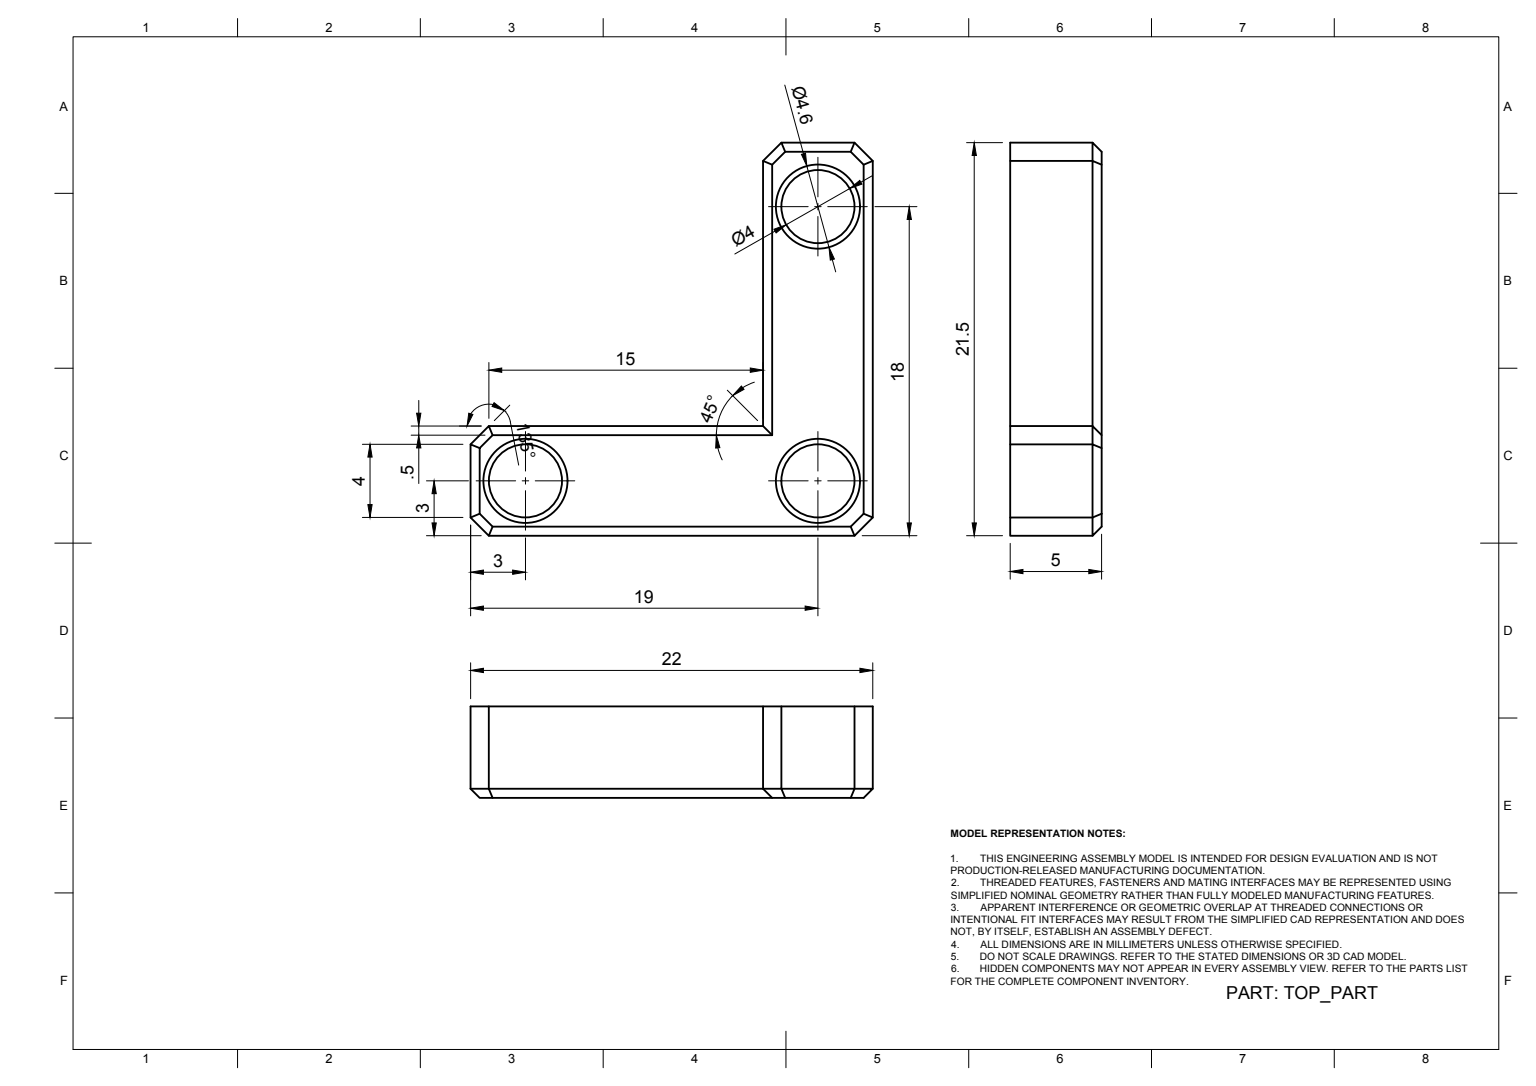
ISO-10303-21;
HEADER;
/* Generated by software containing ST-Developer
 * from STEP Tools, Inc. (www.steptools.com) 
 */

FILE_DESCRIPTION(
/* description */ (''),
/* implementation_level */ '2;1');

FILE_NAME(
/* name */ 'Top_part.step',
/* time_stamp */ '2026-10-04T23:23:09-07:00',
/* author */ (''),
/* organization */ (''),
/* preprocessor_version */ 'ST-DEVELOPER v20.2',
/* originating_system */ 'Autodesk Translation Framework v15.15.0.0',
/* authorisation */ '');

FILE_SCHEMA (('AUTOMOTIVE_DESIGN { 1 0 10303 214 3 1 1 }'));
ENDSEC;

DATA;
#10=MECHANICAL_DESIGN_GEOMETRIC_PRESENTATION_REPRESENTATION('',(#75),#2676);
#56=SHAPE_REPRESENTATION_RELATIONSHIP('SRR','None',#2715,#64);
#64=ADVANCED_BREP_SHAPE_REPRESENTATION('',(#86),#2675);
#75=STYLED_ITEM('',(#2757),#86);
#86=MANIFOLD_SOLID_BREP('Body1',#1486);
#106=CYLINDRICAL_SURFACE('',#1721,2.);
#107=CYLINDRICAL_SURFACE('',#1725,2.);
#108=CYLINDRICAL_SURFACE('',#1753,2.);
#129=FACE_BOUND('',#375,.T.);
#130=FACE_BOUND('',#376,.T.);
#131=FACE_BOUND('',#377,.T.);
#132=FACE_BOUND('',#390,.T.);
#133=FACE_BOUND('',#391,.T.);
#134=FACE_BOUND('',#392,.T.);
#163=PLANE('',#1718);
#164=PLANE('',#1727);
#165=PLANE('',#1728);
#166=PLANE('',#1729);
#167=PLANE('',#1730);
#168=PLANE('',#1731);
#169=PLANE('',#1732);
#170=PLANE('',#1733);
#171=PLANE('',#1734);
#172=PLANE('',#1735);
#173=PLANE('',#1737);
#174=PLANE('',#1738);
#175=PLANE('',#1739);
#176=PLANE('',#1740);
#177=PLANE('',#1741);
#178=PLANE('',#1742);
#179=PLANE('',#1743);
#180=PLANE('',#1744);
#181=PLANE('',#1745);
#182=PLANE('',#1746);
#183=PLANE('',#1747);
#184=PLANE('',#1748);
#185=PLANE('',#1749);
#186=PLANE('',#1750);
#255=FACE_OUTER_BOUND('',#373,.T.);
#256=FACE_OUTER_BOUND('',#374,.T.);
#257=FACE_OUTER_BOUND('',#378,.T.);
#258=FACE_OUTER_BOUND('',#379,.T.);
#259=FACE_OUTER_BOUND('',#380,.T.);
#260=FACE_OUTER_BOUND('',#381,.T.);
#261=FACE_OUTER_BOUND('',#382,.T.);
#262=FACE_OUTER_BOUND('',#383,.T.);
#263=FACE_OUTER_BOUND('',#384,.T.);
#264=FACE_OUTER_BOUND('',#385,.T.);
#265=FACE_OUTER_BOUND('',#386,.T.);
#266=FACE_OUTER_BOUND('',#387,.T.);
#267=FACE_OUTER_BOUND('',#388,.T.);
#268=FACE_OUTER_BOUND('',#389,.T.);
#269=FACE_OUTER_BOUND('',#393,.T.);
#270=FACE_OUTER_BOUND('',#394,.T.);
#271=FACE_OUTER_BOUND('',#395,.T.);
#272=FACE_OUTER_BOUND('',#396,.T.);
#273=FACE_OUTER_BOUND('',#397,.T.);
#274=FACE_OUTER_BOUND('',#398,.T.);
#275=FACE_OUTER_BOUND('',#399,.T.);
#276=FACE_OUTER_BOUND('',#400,.T.);
#277=FACE_OUTER_BOUND('',#401,.T.);
#278=FACE_OUTER_BOUND('',#402,.T.);
#279=FACE_OUTER_BOUND('',#403,.T.);
#280=FACE_OUTER_BOUND('',#404,.T.);
#281=FACE_OUTER_BOUND('',#405,.T.);
#282=FACE_OUTER_BOUND('',#406,.T.);
#283=FACE_OUTER_BOUND('',#407,.T.);
#284=FACE_OUTER_BOUND('',#408,.T.);
#373=EDGE_LOOP('',(#1220,#1221,#1222,#1223));
#374=EDGE_LOOP('',(#1224,#1225,#1226,#1227,#1228,#1229,#1230,#1231,#1232,
#1233,#1234));
#375=EDGE_LOOP('',(#1235));
#376=EDGE_LOOP('',(#1236));
#377=EDGE_LOOP('',(#1237));
#378=EDGE_LOOP('',(#1238,#1239,#1240,#1241));
#379=EDGE_LOOP('',(#1242,#1243,#1244,#1245));
#380=EDGE_LOOP('',(#1246,#1247,#1248,#1249));
#381=EDGE_LOOP('',(#1250,#1251,#1252,#1253));
#382=EDGE_LOOP('',(#1254,#1255,#1256,#1257));
#383=EDGE_LOOP('',(#1258,#1259,#1260,#1261));
#384=EDGE_LOOP('',(#1262,#1263,#1264,#1265));
#385=EDGE_LOOP('',(#1266,#1267,#1268,#1269));
#386=EDGE_LOOP('',(#1270,#1271,#1272,#1273));
#387=EDGE_LOOP('',(#1274,#1275,#1276,#1277));
#388=EDGE_LOOP('',(#1278,#1279,#1280,#1281));
#389=EDGE_LOOP('',(#1282,#1283,#1284,#1285,#1286,#1287,#1288,#1289,#1290,
#1291,#1292));
#390=EDGE_LOOP('',(#1293));
#391=EDGE_LOOP('',(#1294));
#392=EDGE_LOOP('',(#1295));
#393=EDGE_LOOP('',(#1296,#1297,#1298,#1299));
#394=EDGE_LOOP('',(#1300,#1301,#1302,#1303));
#395=EDGE_LOOP('',(#1304,#1305,#1306,#1307));
#396=EDGE_LOOP('',(#1308,#1309,#1310,#1311));
#397=EDGE_LOOP('',(#1312,#1313,#1314,#1315));
#398=EDGE_LOOP('',(#1316,#1317,#1318,#1319));
#399=EDGE_LOOP('',(#1320,#1321,#1322,#1323));
#400=EDGE_LOOP('',(#1324,#1325,#1326,#1327));
#401=EDGE_LOOP('',(#1328,#1329,#1330,#1331));
#402=EDGE_LOOP('',(#1332,#1333,#1334,#1335));
#403=EDGE_LOOP('',(#1336,#1337,#1338,#1339));
#404=EDGE_LOOP('',(#1340,#1341,#1342,#1343));
#405=EDGE_LOOP('',(#1344,#1345,#1346,#1347));
#406=EDGE_LOOP('',(#1348,#1349,#1350,#1351));
#407=EDGE_LOOP('',(#1352,#1353,#1354,#1355));
#408=EDGE_LOOP('',(#1356,#1357,#1358,#1359));
#458=LINE('',#2511,#568);
#459=LINE('',#2516,#569);
#460=LINE('',#2518,#570);
#461=LINE('',#2520,#571);
#462=LINE('',#2522,#572);
#463=LINE('',#2524,#573);
#464=LINE('',#2526,#574);
#465=LINE('',#2528,#575);
#466=LINE('',#2530,#576);
#467=LINE('',#2532,#577);
#468=LINE('',#2534,#578);
#469=LINE('',#2535,#579);
#470=LINE('',#2542,#580);
#471=LINE('',#2547,#581);
#472=LINE('',#2550,#582);
#473=LINE('',#2555,#583);
#474=LINE('',#2556,#584);
#475=LINE('',#2557,#585);
#476=LINE('',#2560,#586);
#477=LINE('',#2561,#587);
#478=LINE('',#2564,#588);
#479=LINE('',#2565,#589);
#480=LINE('',#2568,#590);
#481=LINE('',#2569,#591);
#482=LINE('',#2572,#592);
#483=LINE('',#2574,#593);
#484=LINE('',#2575,#594);
#485=LINE('',#2578,#595);
#486=LINE('',#2579,#596);
#487=LINE('',#2582,#597);
#488=LINE('',#2583,#598);
#489=LINE('',#2586,#599);
#490=LINE('',#2587,#600);
#491=LINE('',#2590,#601);
#492=LINE('',#2592,#602);
#493=LINE('',#2594,#603);
#494=LINE('',#2596,#604);
#495=LINE('',#2598,#605);
#496=LINE('',#2600,#606);
#497=LINE('',#2601,#607);
#498=LINE('',#2606,#608);
#499=LINE('',#2607,#609);
#500=LINE('',#2610,#610);
#501=LINE('',#2612,#611);
#502=LINE('',#2613,#612);
#503=LINE('',#2616,#613);
#504=LINE('',#2617,#614);
#505=LINE('',#2620,#615);
#506=LINE('',#2621,#616);
#507=LINE('',#2624,#617);
#508=LINE('',#2625,#618);
#509=LINE('',#2627,#619);
#510=LINE('',#2629,#620);
#511=LINE('',#2631,#621);
#512=LINE('',#2633,#622);
#513=LINE('',#2635,#623);
#514=LINE('',#2637,#624);
#515=LINE('',#2639,#625);
#516=LINE('',#2641,#626);
#517=LINE('',#2646,#627);
#518=LINE('',#2648,#628);
#568=VECTOR('',#2093,2.15);
#569=VECTOR('',#2098,10.);
#570=VECTOR('',#2099,10.);
#571=VECTOR('',#2100,10.);
#572=VECTOR('',#2101,10.);
#573=VECTOR('',#2102,10.);
#574=VECTOR('',#2103,10.);
#575=VECTOR('',#2104,10.);
#576=VECTOR('',#2105,10.);
#577=VECTOR('',#2106,10.);
#578=VECTOR('',#2107,9.99999999999999);
#579=VECTOR('',#2108,10.);
#580=VECTOR('',#2115,2.);
#581=VECTOR('',#2122,2.15);
#582=VECTOR('',#2125,2.);
#583=VECTOR('',#2130,10.);
#584=VECTOR('',#2131,10.);
#585=VECTOR('',#2132,10.);
#586=VECTOR('',#2135,10.);
#587=VECTOR('',#2136,10.);
#588=VECTOR('',#2139,10.);
#589=VECTOR('',#2140,9.99999999999999);
#590=VECTOR('',#2143,10.);
#591=VECTOR('',#2144,10.);
#592=VECTOR('',#2147,10.);
#593=VECTOR('',#2148,10.);
#594=VECTOR('',#2149,10.);
#595=VECTOR('',#2152,10.);
#596=VECTOR('',#2153,10.);
#597=VECTOR('',#2156,10.);
#598=VECTOR('',#2157,9.99999999999999);
#599=VECTOR('',#2160,10.);
#600=VECTOR('',#2161,10.);
#601=VECTOR('',#2164,10.);
#602=VECTOR('',#2165,10.);
#603=VECTOR('',#2166,10.);
#604=VECTOR('',#2167,10.);
#605=VECTOR('',#2168,10.);
#606=VECTOR('',#2169,10.);
#607=VECTOR('',#2170,10.);
#608=VECTOR('',#2175,10.);
#609=VECTOR('',#2176,10.);
#610=VECTOR('',#2179,10.);
#611=VECTOR('',#2180,10.);
#612=VECTOR('',#2181,10.);
#613=VECTOR('',#2184,10.);
#614=VECTOR('',#2185,10.);
#615=VECTOR('',#2188,10.);
#616=VECTOR('',#2189,10.);
#617=VECTOR('',#2192,10.);
#618=VECTOR('',#2193,10.);
#619=VECTOR('',#2196,10.);
#620=VECTOR('',#2199,10.);
#621=VECTOR('',#2202,10.);
#622=VECTOR('',#2205,10.);
#623=VECTOR('',#2208,10.);
#624=VECTOR('',#2211,10.);
#625=VECTOR('',#2214,10.);
#626=VECTOR('',#2217,10.);
#627=VECTOR('',#2224,2.15);
#628=VECTOR('',#2227,2.);
#691=CIRCLE('',#1716,2.);
#692=CIRCLE('',#1717,2.3);
#693=CIRCLE('',#1719,2.3);
#694=CIRCLE('',#1720,2.3);
#695=CIRCLE('',#1722,2.);
#696=CIRCLE('',#1724,2.);
#697=CIRCLE('',#1726,2.);
#698=CIRCLE('',#1736,2.);
#699=CIRCLE('',#1752,2.);
#775=VERTEX_POINT('',#2508);
#776=VERTEX_POINT('',#2510);
#777=VERTEX_POINT('',#2514);
#778=VERTEX_POINT('',#2515);
#779=VERTEX_POINT('',#2517);
#780=VERTEX_POINT('',#2519);
#781=VERTEX_POINT('',#2521);
#782=VERTEX_POINT('',#2523);
#783=VERTEX_POINT('',#2525);
#784=VERTEX_POINT('',#2527);
#785=VERTEX_POINT('',#2529);
#786=VERTEX_POINT('',#2531);
#787=VERTEX_POINT('',#2533);
#788=VERTEX_POINT('',#2536);
#789=VERTEX_POINT('',#2538);
#790=VERTEX_POINT('',#2541);
#791=VERTEX_POINT('',#2545);
#792=VERTEX_POINT('',#2549);
#793=VERTEX_POINT('',#2553);
#794=VERTEX_POINT('',#2554);
#795=VERTEX_POINT('',#2559);
#796=VERTEX_POINT('',#2563);
#797=VERTEX_POINT('',#2567);
#798=VERTEX_POINT('',#2571);
#799=VERTEX_POINT('',#2573);
#800=VERTEX_POINT('',#2577);
#801=VERTEX_POINT('',#2581);
#802=VERTEX_POINT('',#2585);
#803=VERTEX_POINT('',#2589);
#804=VERTEX_POINT('',#2591);
#805=VERTEX_POINT('',#2593);
#806=VERTEX_POINT('',#2595);
#807=VERTEX_POINT('',#2597);
#808=VERTEX_POINT('',#2599);
#809=VERTEX_POINT('',#2602);
#810=VERTEX_POINT('',#2605);
#811=VERTEX_POINT('',#2609);
#812=VERTEX_POINT('',#2611);
#813=VERTEX_POINT('',#2615);
#814=VERTEX_POINT('',#2619);
#815=VERTEX_POINT('',#2623);
#816=VERTEX_POINT('',#2644);
#928=EDGE_CURVE('',#775,#775,#691,.T.);
#929=EDGE_CURVE('',#775,#776,#458,.T.);
#930=EDGE_CURVE('',#776,#776,#692,.T.);
#931=EDGE_CURVE('',#777,#778,#459,.T.);
#932=EDGE_CURVE('',#779,#777,#460,.T.);
#933=EDGE_CURVE('',#780,#779,#461,.T.);
#934=EDGE_CURVE('',#781,#780,#462,.T.);
#935=EDGE_CURVE('',#782,#781,#463,.T.);
#936=EDGE_CURVE('',#783,#782,#464,.T.);
#937=EDGE_CURVE('',#784,#783,#465,.T.);
#938=EDGE_CURVE('',#785,#784,#466,.T.);
#939=EDGE_CURVE('',#786,#785,#467,.T.);
#940=EDGE_CURVE('',#787,#786,#468,.T.);
#941=EDGE_CURVE('',#778,#787,#469,.T.);
#942=EDGE_CURVE('',#788,#788,#693,.T.);
#943=EDGE_CURVE('',#789,#789,#694,.T.);
#944=EDGE_CURVE('',#775,#790,#470,.T.);
#945=EDGE_CURVE('',#790,#790,#695,.T.);
#946=EDGE_CURVE('',#791,#791,#696,.T.);
#947=EDGE_CURVE('',#791,#788,#471,.T.);
#948=EDGE_CURVE('',#791,#792,#472,.T.);
#949=EDGE_CURVE('',#792,#792,#697,.T.);
#950=EDGE_CURVE('',#793,#794,#473,.T.);
#951=EDGE_CURVE('',#794,#777,#474,.T.);
#952=EDGE_CURVE('',#778,#793,#475,.T.);
#953=EDGE_CURVE('',#787,#795,#476,.T.);
#954=EDGE_CURVE('',#795,#793,#477,.T.);
#955=EDGE_CURVE('',#786,#796,#478,.T.);
#956=EDGE_CURVE('',#796,#795,#479,.T.);
#957=EDGE_CURVE('',#785,#797,#480,.F.);
#958=EDGE_CURVE('',#797,#796,#481,.T.);
#959=EDGE_CURVE('',#793,#798,#482,.T.);
#960=EDGE_CURVE('',#798,#799,#483,.T.);
#961=EDGE_CURVE('',#799,#794,#484,.T.);
#962=EDGE_CURVE('',#800,#795,#485,.T.);
#963=EDGE_CURVE('',#800,#798,#486,.T.);
#964=EDGE_CURVE('',#796,#801,#487,.T.);
#965=EDGE_CURVE('',#801,#800,#488,.T.);
#966=EDGE_CURVE('',#802,#797,#489,.T.);
#967=EDGE_CURVE('',#802,#801,#490,.F.);
#968=EDGE_CURVE('',#803,#802,#491,.T.);
#969=EDGE_CURVE('',#804,#803,#492,.T.);
#970=EDGE_CURVE('',#804,#805,#493,.T.);
#971=EDGE_CURVE('',#806,#805,#494,.T.);
#972=EDGE_CURVE('',#807,#806,#495,.T.);
#973=EDGE_CURVE('',#808,#807,#496,.T.);
#974=EDGE_CURVE('',#799,#808,#497,.F.);
#975=EDGE_CURVE('',#809,#809,#698,.T.);
#976=EDGE_CURVE('',#810,#797,#498,.T.);
#977=EDGE_CURVE('',#784,#810,#499,.T.);
#978=EDGE_CURVE('',#782,#811,#500,.T.);
#979=EDGE_CURVE('',#811,#812,#501,.T.);
#980=EDGE_CURVE('',#812,#783,#502,.T.);
#981=EDGE_CURVE('',#781,#813,#503,.T.);
#982=EDGE_CURVE('',#813,#811,#504,.T.);
#983=EDGE_CURVE('',#780,#814,#505,.T.);
#984=EDGE_CURVE('',#814,#813,#506,.T.);
#985=EDGE_CURVE('',#779,#815,#507,.T.);
#986=EDGE_CURVE('',#815,#814,#508,.T.);
#987=EDGE_CURVE('',#794,#815,#509,.T.);
#988=EDGE_CURVE('',#812,#810,#510,.T.);
#989=EDGE_CURVE('',#803,#810,#511,.T.);
#990=EDGE_CURVE('',#812,#804,#512,.T.);
#991=EDGE_CURVE('',#805,#811,#513,.T.);
#992=EDGE_CURVE('',#813,#806,#514,.T.);
#993=EDGE_CURVE('',#807,#814,#515,.T.);
#994=EDGE_CURVE('',#815,#808,#516,.T.);
#995=EDGE_CURVE('',#816,#816,#699,.T.);
#996=EDGE_CURVE('',#816,#789,#517,.T.);
#997=EDGE_CURVE('',#816,#809,#518,.T.);
#1220=ORIENTED_EDGE('',*,*,#928,.T.);
#1221=ORIENTED_EDGE('',*,*,#929,.T.);
#1222=ORIENTED_EDGE('',*,*,#930,.T.);
#1223=ORIENTED_EDGE('',*,*,#929,.F.);
#1224=ORIENTED_EDGE('',*,*,#931,.F.);
#1225=ORIENTED_EDGE('',*,*,#932,.F.);
#1226=ORIENTED_EDGE('',*,*,#933,.F.);
#1227=ORIENTED_EDGE('',*,*,#934,.F.);
#1228=ORIENTED_EDGE('',*,*,#935,.F.);
#1229=ORIENTED_EDGE('',*,*,#936,.F.);
#1230=ORIENTED_EDGE('',*,*,#937,.F.);
#1231=ORIENTED_EDGE('',*,*,#938,.F.);
#1232=ORIENTED_EDGE('',*,*,#939,.F.);
#1233=ORIENTED_EDGE('',*,*,#940,.F.);
#1234=ORIENTED_EDGE('',*,*,#941,.F.);
#1235=ORIENTED_EDGE('',*,*,#942,.F.);
#1236=ORIENTED_EDGE('',*,*,#943,.F.);
#1237=ORIENTED_EDGE('',*,*,#930,.F.);
#1238=ORIENTED_EDGE('',*,*,#928,.F.);
#1239=ORIENTED_EDGE('',*,*,#944,.T.);
#1240=ORIENTED_EDGE('',*,*,#945,.F.);
#1241=ORIENTED_EDGE('',*,*,#944,.F.);
#1242=ORIENTED_EDGE('',*,*,#946,.T.);
#1243=ORIENTED_EDGE('',*,*,#947,.T.);
#1244=ORIENTED_EDGE('',*,*,#942,.T.);
#1245=ORIENTED_EDGE('',*,*,#947,.F.);
#1246=ORIENTED_EDGE('',*,*,#946,.F.);
#1247=ORIENTED_EDGE('',*,*,#948,.T.);
#1248=ORIENTED_EDGE('',*,*,#949,.F.);
#1249=ORIENTED_EDGE('',*,*,#948,.F.);
#1250=ORIENTED_EDGE('',*,*,#950,.T.);
#1251=ORIENTED_EDGE('',*,*,#951,.T.);
#1252=ORIENTED_EDGE('',*,*,#931,.T.);
#1253=ORIENTED_EDGE('',*,*,#952,.T.);
#1254=ORIENTED_EDGE('',*,*,#941,.T.);
#1255=ORIENTED_EDGE('',*,*,#953,.T.);
#1256=ORIENTED_EDGE('',*,*,#954,.T.);
#1257=ORIENTED_EDGE('',*,*,#952,.F.);
#1258=ORIENTED_EDGE('',*,*,#940,.T.);
#1259=ORIENTED_EDGE('',*,*,#955,.T.);
#1260=ORIENTED_EDGE('',*,*,#956,.T.);
#1261=ORIENTED_EDGE('',*,*,#953,.F.);
#1262=ORIENTED_EDGE('',*,*,#939,.T.);
#1263=ORIENTED_EDGE('',*,*,#957,.T.);
#1264=ORIENTED_EDGE('',*,*,#958,.T.);
#1265=ORIENTED_EDGE('',*,*,#955,.F.);
#1266=ORIENTED_EDGE('',*,*,#950,.F.);
#1267=ORIENTED_EDGE('',*,*,#959,.T.);
#1268=ORIENTED_EDGE('',*,*,#960,.T.);
#1269=ORIENTED_EDGE('',*,*,#961,.T.);
#1270=ORIENTED_EDGE('',*,*,#954,.F.);
#1271=ORIENTED_EDGE('',*,*,#962,.F.);
#1272=ORIENTED_EDGE('',*,*,#963,.T.);
#1273=ORIENTED_EDGE('',*,*,#959,.F.);
#1274=ORIENTED_EDGE('',*,*,#956,.F.);
#1275=ORIENTED_EDGE('',*,*,#964,.T.);
#1276=ORIENTED_EDGE('',*,*,#965,.T.);
#1277=ORIENTED_EDGE('',*,*,#962,.T.);
#1278=ORIENTED_EDGE('',*,*,#958,.F.);
#1279=ORIENTED_EDGE('',*,*,#966,.F.);
#1280=ORIENTED_EDGE('',*,*,#967,.T.);
#1281=ORIENTED_EDGE('',*,*,#964,.F.);
#1282=ORIENTED_EDGE('',*,*,#965,.F.);
#1283=ORIENTED_EDGE('',*,*,#967,.F.);
#1284=ORIENTED_EDGE('',*,*,#968,.F.);
#1285=ORIENTED_EDGE('',*,*,#969,.F.);
#1286=ORIENTED_EDGE('',*,*,#970,.T.);
#1287=ORIENTED_EDGE('',*,*,#971,.F.);
#1288=ORIENTED_EDGE('',*,*,#972,.F.);
#1289=ORIENTED_EDGE('',*,*,#973,.F.);
#1290=ORIENTED_EDGE('',*,*,#974,.F.);
#1291=ORIENTED_EDGE('',*,*,#960,.F.);
#1292=ORIENTED_EDGE('',*,*,#963,.F.);
#1293=ORIENTED_EDGE('',*,*,#945,.T.);
#1294=ORIENTED_EDGE('',*,*,#949,.T.);
#1295=ORIENTED_EDGE('',*,*,#975,.T.);
#1296=ORIENTED_EDGE('',*,*,#976,.T.);
#1297=ORIENTED_EDGE('',*,*,#957,.F.);
#1298=ORIENTED_EDGE('',*,*,#938,.T.);
#1299=ORIENTED_EDGE('',*,*,#977,.T.);
#1300=ORIENTED_EDGE('',*,*,#936,.T.);
#1301=ORIENTED_EDGE('',*,*,#978,.T.);
#1302=ORIENTED_EDGE('',*,*,#979,.T.);
#1303=ORIENTED_EDGE('',*,*,#980,.T.);
#1304=ORIENTED_EDGE('',*,*,#935,.T.);
#1305=ORIENTED_EDGE('',*,*,#981,.T.);
#1306=ORIENTED_EDGE('',*,*,#982,.T.);
#1307=ORIENTED_EDGE('',*,*,#978,.F.);
#1308=ORIENTED_EDGE('',*,*,#934,.T.);
#1309=ORIENTED_EDGE('',*,*,#983,.T.);
#1310=ORIENTED_EDGE('',*,*,#984,.T.);
#1311=ORIENTED_EDGE('',*,*,#981,.F.);
#1312=ORIENTED_EDGE('',*,*,#933,.T.);
#1313=ORIENTED_EDGE('',*,*,#985,.T.);
#1314=ORIENTED_EDGE('',*,*,#986,.T.);
#1315=ORIENTED_EDGE('',*,*,#983,.F.);
#1316=ORIENTED_EDGE('',*,*,#951,.F.);
#1317=ORIENTED_EDGE('',*,*,#987,.T.);
#1318=ORIENTED_EDGE('',*,*,#985,.F.);
#1319=ORIENTED_EDGE('',*,*,#932,.T.);
#1320=ORIENTED_EDGE('',*,*,#937,.T.);
#1321=ORIENTED_EDGE('',*,*,#980,.F.);
#1322=ORIENTED_EDGE('',*,*,#988,.T.);
#1323=ORIENTED_EDGE('',*,*,#977,.F.);
#1324=ORIENTED_EDGE('',*,*,#976,.F.);
#1325=ORIENTED_EDGE('',*,*,#989,.F.);
#1326=ORIENTED_EDGE('',*,*,#968,.T.);
#1327=ORIENTED_EDGE('',*,*,#966,.T.);
#1328=ORIENTED_EDGE('',*,*,#988,.F.);
#1329=ORIENTED_EDGE('',*,*,#990,.T.);
#1330=ORIENTED_EDGE('',*,*,#969,.T.);
#1331=ORIENTED_EDGE('',*,*,#989,.T.);
#1332=ORIENTED_EDGE('',*,*,#979,.F.);
#1333=ORIENTED_EDGE('',*,*,#991,.F.);
#1334=ORIENTED_EDGE('',*,*,#970,.F.);
#1335=ORIENTED_EDGE('',*,*,#990,.F.);
#1336=ORIENTED_EDGE('',*,*,#982,.F.);
#1337=ORIENTED_EDGE('',*,*,#992,.T.);
#1338=ORIENTED_EDGE('',*,*,#971,.T.);
#1339=ORIENTED_EDGE('',*,*,#991,.T.);
#1340=ORIENTED_EDGE('',*,*,#984,.F.);
#1341=ORIENTED_EDGE('',*,*,#993,.F.);
#1342=ORIENTED_EDGE('',*,*,#972,.T.);
#1343=ORIENTED_EDGE('',*,*,#992,.F.);
#1344=ORIENTED_EDGE('',*,*,#986,.F.);
#1345=ORIENTED_EDGE('',*,*,#994,.T.);
#1346=ORIENTED_EDGE('',*,*,#973,.T.);
#1347=ORIENTED_EDGE('',*,*,#993,.T.);
#1348=ORIENTED_EDGE('',*,*,#987,.F.);
#1349=ORIENTED_EDGE('',*,*,#961,.F.);
#1350=ORIENTED_EDGE('',*,*,#974,.T.);
#1351=ORIENTED_EDGE('',*,*,#994,.F.);
#1352=ORIENTED_EDGE('',*,*,#995,.T.);
#1353=ORIENTED_EDGE('',*,*,#996,.T.);
#1354=ORIENTED_EDGE('',*,*,#943,.T.);
#1355=ORIENTED_EDGE('',*,*,#996,.F.);
#1356=ORIENTED_EDGE('',*,*,#995,.F.);
#1357=ORIENTED_EDGE('',*,*,#997,.T.);
#1358=ORIENTED_EDGE('',*,*,#975,.F.);
#1359=ORIENTED_EDGE('',*,*,#997,.F.);
#1375=CONICAL_SURFACE('',#1715,2.15,0.785398163397448);
#1376=CONICAL_SURFACE('',#1723,2.15,0.785398163397448);
#1377=CONICAL_SURFACE('',#1751,2.15,0.785398163397448);
#1446=ADVANCED_FACE('',(#255),#1375,.F.);
#1447=ADVANCED_FACE('',(#256,#129,#130,#131),#163,.T.);
#1448=ADVANCED_FACE('',(#257),#106,.F.);
#1449=ADVANCED_FACE('',(#258),#1376,.F.);
#1450=ADVANCED_FACE('',(#259),#107,.F.);
#1451=ADVANCED_FACE('',(#260),#164,.T.);
#1452=ADVANCED_FACE('',(#261),#165,.T.);
#1453=ADVANCED_FACE('',(#262),#166,.T.);
#1454=ADVANCED_FACE('',(#263),#167,.T.);
#1455=ADVANCED_FACE('',(#264),#168,.T.);
#1456=ADVANCED_FACE('',(#265),#169,.T.);
#1457=ADVANCED_FACE('',(#266),#170,.T.);
#1458=ADVANCED_FACE('',(#267),#171,.T.);
#1459=ADVANCED_FACE('',(#268,#132,#133,#134),#172,.F.);
#1460=ADVANCED_FACE('',(#269),#173,.T.);
#1461=ADVANCED_FACE('',(#270),#174,.T.);
#1462=ADVANCED_FACE('',(#271),#175,.T.);
#1463=ADVANCED_FACE('',(#272),#176,.T.);
#1464=ADVANCED_FACE('',(#273),#177,.T.);
#1465=ADVANCED_FACE('',(#274),#178,.T.);
#1466=ADVANCED_FACE('',(#275),#179,.T.);
#1467=ADVANCED_FACE('',(#276),#180,.T.);
#1468=ADVANCED_FACE('',(#277),#181,.T.);
#1469=ADVANCED_FACE('',(#278),#182,.T.);
#1470=ADVANCED_FACE('',(#279),#183,.T.);
#1471=ADVANCED_FACE('',(#280),#184,.T.);
#1472=ADVANCED_FACE('',(#281),#185,.T.);
#1473=ADVANCED_FACE('',(#282),#186,.T.);
#1474=ADVANCED_FACE('',(#283),#1377,.F.);
#1475=ADVANCED_FACE('',(#284),#108,.F.);
#1486=CLOSED_SHELL('',(#1446,#1447,#1448,#1449,#1450,#1451,#1452,#1453,
#1454,#1455,#1456,#1457,#1458,#1459,#1460,#1461,#1462,#1463,#1464,#1465,
#1466,#1467,#1468,#1469,#1470,#1471,#1472,#1473,#1474,#1475));
#1714=AXIS2_PLACEMENT_3D('',#2506,#2087,#2088);
#1715=AXIS2_PLACEMENT_3D('',#2507,#2089,#2090);
#1716=AXIS2_PLACEMENT_3D('',#2509,#2091,#2092);
#1717=AXIS2_PLACEMENT_3D('',#2512,#2094,#2095);
#1718=AXIS2_PLACEMENT_3D('',#2513,#2096,#2097);
#1719=AXIS2_PLACEMENT_3D('',#2537,#2109,#2110);
#1720=AXIS2_PLACEMENT_3D('',#2539,#2111,#2112);
#1721=AXIS2_PLACEMENT_3D('',#2540,#2113,#2114);
#1722=AXIS2_PLACEMENT_3D('',#2543,#2116,#2117);
#1723=AXIS2_PLACEMENT_3D('',#2544,#2118,#2119);
#1724=AXIS2_PLACEMENT_3D('',#2546,#2120,#2121);
#1725=AXIS2_PLACEMENT_3D('',#2548,#2123,#2124);
#1726=AXIS2_PLACEMENT_3D('',#2551,#2126,#2127);
#1727=AXIS2_PLACEMENT_3D('',#2552,#2128,#2129);
#1728=AXIS2_PLACEMENT_3D('',#2558,#2133,#2134);
#1729=AXIS2_PLACEMENT_3D('',#2562,#2137,#2138);
#1730=AXIS2_PLACEMENT_3D('',#2566,#2141,#2142);
#1731=AXIS2_PLACEMENT_3D('',#2570,#2145,#2146);
#1732=AXIS2_PLACEMENT_3D('',#2576,#2150,#2151);
#1733=AXIS2_PLACEMENT_3D('',#2580,#2154,#2155);
#1734=AXIS2_PLACEMENT_3D('',#2584,#2158,#2159);
#1735=AXIS2_PLACEMENT_3D('',#2588,#2162,#2163);
#1736=AXIS2_PLACEMENT_3D('',#2603,#2171,#2172);
#1737=AXIS2_PLACEMENT_3D('',#2604,#2173,#2174);
#1738=AXIS2_PLACEMENT_3D('',#2608,#2177,#2178);
#1739=AXIS2_PLACEMENT_3D('',#2614,#2182,#2183);
#1740=AXIS2_PLACEMENT_3D('',#2618,#2186,#2187);
#1741=AXIS2_PLACEMENT_3D('',#2622,#2190,#2191);
#1742=AXIS2_PLACEMENT_3D('',#2626,#2194,#2195);
#1743=AXIS2_PLACEMENT_3D('',#2628,#2197,#2198);
#1744=AXIS2_PLACEMENT_3D('',#2630,#2200,#2201);
#1745=AXIS2_PLACEMENT_3D('',#2632,#2203,#2204);
#1746=AXIS2_PLACEMENT_3D('',#2634,#2206,#2207);
#1747=AXIS2_PLACEMENT_3D('',#2636,#2209,#2210);
#1748=AXIS2_PLACEMENT_3D('',#2638,#2212,#2213);
#1749=AXIS2_PLACEMENT_3D('',#2640,#2215,#2216);
#1750=AXIS2_PLACEMENT_3D('',#2642,#2218,#2219);
#1751=AXIS2_PLACEMENT_3D('',#2643,#2220,#2221);
#1752=AXIS2_PLACEMENT_3D('',#2645,#2222,#2223);
#1753=AXIS2_PLACEMENT_3D('',#2647,#2225,#2226);
#2087=DIRECTION('axis',(0.,0.,1.));
#2088=DIRECTION('refdir',(1.,0.,0.));
#2089=DIRECTION('center_axis',(0.,0.,1.));
#2090=DIRECTION('ref_axis',(-1.,0.,0.));
#2091=DIRECTION('center_axis',(0.,0.,-1.));
#2092=DIRECTION('ref_axis',(-1.,0.,0.));
#2093=DIRECTION('',(0.707106781186547,8.65956056235493E-17,0.707106781186548));
#2094=DIRECTION('center_axis',(0.,0.,1.));
#2095=DIRECTION('ref_axis',(-1.,0.,0.));
#2096=DIRECTION('center_axis',(0.,0.,1.));
#2097=DIRECTION('ref_axis',(1.,0.,0.));
#2098=DIRECTION('',(-0.707106781186548,0.707106781186547,0.));
#2099=DIRECTION('',(-1.,0.,0.));
#2100=DIRECTION('',(-0.707106781186548,-0.707106781186547,0.));
#2101=DIRECTION('',(0.,-1.,0.));
#2102=DIRECTION('',(0.707106781186547,-0.707106781186547,0.));
#2103=DIRECTION('',(1.,0.,0.));
#2104=DIRECTION('',(0.707106781186547,0.707106781186548,0.));
#2105=DIRECTION('',(0.,1.,0.));
#2106=DIRECTION('',(1.,0.,0.));
#2107=DIRECTION('',(0.707106781186548,0.707106781186547,0.));
#2108=DIRECTION('',(0.,1.,0.));
#2109=DIRECTION('center_axis',(0.,0.,1.));
#2110=DIRECTION('ref_axis',(-1.,0.,0.));
#2111=DIRECTION('center_axis',(0.,0.,1.));
#2112=DIRECTION('ref_axis',(-1.,0.,0.));
#2113=DIRECTION('center_axis',(0.,0.,-1.));
#2114=DIRECTION('ref_axis',(-1.,0.,0.));
#2115=DIRECTION('',(0.,0.,-1.));
#2116=DIRECTION('center_axis',(0.,0.,1.));
#2117=DIRECTION('ref_axis',(-1.,0.,0.));
#2118=DIRECTION('center_axis',(0.,0.,1.));
#2119=DIRECTION('ref_axis',(-1.,0.,0.));
#2120=DIRECTION('center_axis',(0.,0.,-1.));
#2121=DIRECTION('ref_axis',(-1.,0.,0.));
#2122=DIRECTION('',(0.707106781186547,8.65956056235493E-17,0.707106781186548));
#2123=DIRECTION('center_axis',(0.,0.,-1.));
#2124=DIRECTION('ref_axis',(-1.,0.,0.));
#2125=DIRECTION('',(0.,0.,-1.));
#2126=DIRECTION('center_axis',(0.,0.,1.));
#2127=DIRECTION('ref_axis',(-1.,0.,0.));
#2128=DIRECTION('center_axis',(-0.500000000000001,-0.500000000000001,0.707106781186546));
#2129=DIRECTION('ref_axis',(0.816496580927725,-1.47935320064922E-16,0.577350269189627));
#2130=DIRECTION('',(0.707106781186548,-0.707106781186547,0.));
#2131=DIRECTION('',(0.281084637714816,0.678598344545848,0.678598344545848));
#2132=DIRECTION('',(-0.678598344545848,-0.281084637714818,-0.678598344545848));
#2133=DIRECTION('center_axis',(-0.707106781186548,0.,0.707106781186548));
#2134=DIRECTION('ref_axis',(0.707106781186548,0.,0.707106781186548));
#2135=DIRECTION('',(-0.678598344545847,0.281084637714821,-0.678598344545847));
#2136=DIRECTION('',(0.,-1.,0.));
#2137=DIRECTION('center_axis',(-0.5,0.500000000000001,0.707106781186547));
#2138=DIRECTION('ref_axis',(0.816496580927726,1.11022302462516E-16,0.577350269189626));
#2139=DIRECTION('',(-0.281084637714819,0.678598344545847,-0.678598344545848));
#2140=DIRECTION('',(-0.707106781186548,-0.707106781186547,0.));
#2141=DIRECTION('center_axis',(0.,0.707106781186548,0.707106781186547));
#2142=DIRECTION('ref_axis',(1.,0.,0.));
#2143=DIRECTION('',(0.577350269189626,-0.577350269189625,0.577350269189626));
#2144=DIRECTION('',(-1.,0.,0.));
#2145=DIRECTION('center_axis',(-0.707106781186547,-0.707106781186548,0.));
#2146=DIRECTION('ref_axis',(0.,0.,1.));
#2147=DIRECTION('',(0.,0.,-1.));
#2148=DIRECTION('',(0.707106781186548,-0.707106781186547,0.));
#2149=DIRECTION('',(0.,0.,1.));
#2150=DIRECTION('center_axis',(-1.,0.,0.));
#2151=DIRECTION('ref_axis',(0.,-1.,0.));
#2152=DIRECTION('',(0.,0.,1.));
#2153=DIRECTION('',(0.,-1.,0.));
#2154=DIRECTION('center_axis',(-0.707106781186547,0.707106781186549,0.));
#2155=DIRECTION('ref_axis',(0.,0.,1.));
#2156=DIRECTION('',(0.,0.,-1.));
#2157=DIRECTION('',(-0.707106781186548,-0.707106781186547,0.));
#2158=DIRECTION('center_axis',(0.,1.,0.));
#2159=DIRECTION('ref_axis',(-1.,0.,0.));
#2160=DIRECTION('',(0.,0.,1.));
#2161=DIRECTION('',(1.,0.,0.));
#2162=DIRECTION('center_axis',(0.,0.,1.));
#2163=DIRECTION('ref_axis',(1.,0.,0.));
#2164=DIRECTION('',(0.,-1.,0.));
#2165=DIRECTION('',(-0.707106781186547,-0.707106781186548,0.));
#2166=DIRECTION('',(1.,0.,0.));
#2167=DIRECTION('',(-0.707106781186547,0.707106781186547,0.));
#2168=DIRECTION('',(0.,1.,0.));
#2169=DIRECTION('',(0.707106781186548,0.707106781186547,0.));
#2170=DIRECTION('',(-1.,0.,0.));
#2171=DIRECTION('center_axis',(0.,0.,1.));
#2172=DIRECTION('ref_axis',(-1.,0.,0.));
#2173=DIRECTION('center_axis',(-0.707106781186548,0.,0.707106781186548));
#2174=DIRECTION('ref_axis',(0.707106781186548,0.,0.707106781186548));
#2175=DIRECTION('',(0.,-1.,0.));
#2176=DIRECTION('',(-0.678598344545848,0.281084637714819,-0.678598344545847));
#2177=DIRECTION('center_axis',(0.,0.707106781186548,0.707106781186548));
#2178=DIRECTION('ref_axis',(1.,0.,0.));
#2179=DIRECTION('',(0.281084637714818,0.678598344545848,-0.678598344545848));
#2180=DIRECTION('',(-1.,0.,0.));
#2181=DIRECTION('',(0.281084637714822,-0.678598344545847,0.678598344545847));
#2182=DIRECTION('center_axis',(0.500000000000001,0.500000000000001,0.707106781186547));
#2183=DIRECTION('ref_axis',(0.816496580927725,1.16630067516701E-16,-0.577350269189627));
#2184=DIRECTION('',(0.678598344545847,0.281084637714819,-0.678598344545847));
#2185=DIRECTION('',(-0.707106781186547,0.707106781186547,0.));
#2186=DIRECTION('center_axis',(0.707106781186548,0.,0.707106781186548));
#2187=DIRECTION('ref_axis',(0.707106781186548,0.,-0.707106781186548));
#2188=DIRECTION('',(0.678598344545847,-0.281084637714821,-0.678598344545847));
#2189=DIRECTION('',(0.,1.,0.));
#2190=DIRECTION('center_axis',(0.5,-0.500000000000001,0.707106781186547));
#2191=DIRECTION('ref_axis',(0.816496580927726,1.11022302462516E-16,-0.577350269189626));
#2192=DIRECTION('',(0.281084637714819,-0.678598344545847,-0.678598344545847));
#2193=DIRECTION('',(0.707106781186548,0.707106781186547,0.));
#2194=DIRECTION('center_axis',(0.,-0.707106781186548,0.707106781186548));
#2195=DIRECTION('ref_axis',(1.,0.,0.));
#2196=DIRECTION('',(1.,0.,0.));
#2197=DIRECTION('center_axis',(-0.500000000000001,0.5,0.707106781186547));
#2198=DIRECTION('ref_axis',(0.816496580927725,-1.19433950043794E-16,0.577350269189627));
#2199=DIRECTION('',(-0.707106781186547,-0.707106781186548,0.));
#2200=DIRECTION('center_axis',(-1.,0.,0.));
#2201=DIRECTION('ref_axis',(0.,-1.,0.));
#2202=DIRECTION('',(0.,0.,1.));
#2203=DIRECTION('center_axis',(-0.707106781186548,0.707106781186547,0.));
#2204=DIRECTION('ref_axis',(0.,0.,1.));
#2205=DIRECTION('',(0.,0.,-1.));
#2206=DIRECTION('center_axis',(0.,1.,0.));
#2207=DIRECTION('ref_axis',(-1.,0.,0.));
#2208=DIRECTION('',(0.,0.,1.));
#2209=DIRECTION('center_axis',(0.707106781186548,0.707106781186548,0.));
#2210=DIRECTION('ref_axis',(0.,0.,-1.));
#2211=DIRECTION('',(0.,0.,-1.));
#2212=DIRECTION('center_axis',(1.,0.,0.));
#2213=DIRECTION('ref_axis',(0.,1.,0.));
#2214=DIRECTION('',(0.,0.,1.));
#2215=DIRECTION('center_axis',(0.707106781186547,-0.707106781186548,0.));
#2216=DIRECTION('ref_axis',(0.,0.,-1.));
#2217=DIRECTION('',(0.,0.,-1.));
#2218=DIRECTION('center_axis',(0.,-1.,0.));
#2219=DIRECTION('ref_axis',(1.,0.,0.));
#2220=DIRECTION('center_axis',(0.,0.,1.));
#2221=DIRECTION('ref_axis',(-1.,0.,0.));
#2222=DIRECTION('center_axis',(0.,0.,-1.));
#2223=DIRECTION('ref_axis',(-1.,0.,0.));
#2224=DIRECTION('',(0.707106781186547,8.65956056235493E-17,0.707106781186548));
#2225=DIRECTION('center_axis',(0.,0.,-1.));
#2226=DIRECTION('ref_axis',(-1.,0.,0.));
#2227=DIRECTION('',(0.,0.,-1.));
#2506=CARTESIAN_POINT('',(0.,0.,0.));
#2507=CARTESIAN_POINT('Origin',(-8.,-7.5,12.35));
#2508=CARTESIAN_POINT('',(-6.,-7.5,12.2));
#2509=CARTESIAN_POINT('Origin',(-8.,-7.5,12.2));
#2510=CARTESIAN_POINT('',(-5.7,-7.5,12.5));
#2511=CARTESIAN_POINT('',(-5.85,-7.5,12.35));
#2512=CARTESIAN_POINT('Origin',(-8.,-7.5,12.5));
#2513=CARTESIAN_POINT('Origin',(0.,0.,12.5));
#2514=CARTESIAN_POINT('',(-9.79289321881345,-10.,12.5));
#2515=CARTESIAN_POINT('',(-10.5,-9.29289321881345,12.5));
#2516=CARTESIAN_POINT('',(-10.0214466094067,-9.77144660940673,12.5));
#2517=CARTESIAN_POINT('',(9.79289321881345,-10.,12.5));
#2518=CARTESIAN_POINT('',(-5.5,-10.,12.5));
#2519=CARTESIAN_POINT('',(10.5,-9.29289321881345,12.5));
#2520=CARTESIAN_POINT('',(10.0214466094067,-9.77144660940673,12.5));
#2521=CARTESIAN_POINT('',(10.5,9.79289321881345,12.5));
#2522=CARTESIAN_POINT('',(10.5,-5.5,12.5));
#2523=CARTESIAN_POINT('',(9.79289321881345,10.5,12.5));
#2524=CARTESIAN_POINT('',(10.1464466094067,10.1464466094067,12.5));
#2525=CARTESIAN_POINT('',(6.20710678118655,10.5,12.5));
#2526=CARTESIAN_POINT('',(5.5,10.5,12.5));
#2527=CARTESIAN_POINT('',(5.5,9.79289321881345,12.5));
#2528=CARTESIAN_POINT('',(1.85355339059327,6.14644660940672,12.5));
#2529=CARTESIAN_POINT('',(5.5,-5.,12.5));
#2530=CARTESIAN_POINT('',(5.5,5.5,12.5));
#2531=CARTESIAN_POINT('',(-9.79289321881345,-5.,12.5));
#2532=CARTESIAN_POINT('',(2.5,-5.,12.5));
#2533=CARTESIAN_POINT('',(-10.5,-5.70710678118654,12.5));
#2534=CARTESIAN_POINT('',(-6.27144660940672,-1.47855339059328,12.5));
#2535=CARTESIAN_POINT('',(-10.5,-2.5,12.5));
#2536=CARTESIAN_POINT('',(10.3,-7.5,12.5));
#2537=CARTESIAN_POINT('Origin',(8.,-7.5,12.5));
#2538=CARTESIAN_POINT('',(10.3,7.5,12.5));
#2539=CARTESIAN_POINT('Origin',(8.,7.5,12.5));
#2540=CARTESIAN_POINT('Origin',(-8.,-7.5,12.5));
#2541=CARTESIAN_POINT('',(-6.,-7.5,7.5));
#2542=CARTESIAN_POINT('',(-6.,-7.5,12.5));
#2543=CARTESIAN_POINT('Origin',(-8.,-7.5,7.5));
#2544=CARTESIAN_POINT('Origin',(8.,-7.5,12.35));
#2545=CARTESIAN_POINT('',(10.,-7.5,12.2));
#2546=CARTESIAN_POINT('Origin',(8.,-7.5,12.2));
#2547=CARTESIAN_POINT('',(10.15,-7.5,12.35));
#2548=CARTESIAN_POINT('Origin',(8.,-7.5,12.5));
#2549=CARTESIAN_POINT('',(10.,-7.5,7.5));
#2550=CARTESIAN_POINT('',(10.,-7.5,12.5));
#2551=CARTESIAN_POINT('Origin',(8.,-7.5,7.5));
#2552=CARTESIAN_POINT('Origin',(-10.1982233047034,-9.94822330470336,12.25));
#2553=CARTESIAN_POINT('',(-11.,-9.5,12.));
#2554=CARTESIAN_POINT('',(-10.,-10.5,12.));
#2555=CARTESIAN_POINT('',(-10.375,-10.125,12.));
#2556=CARTESIAN_POINT('',(-9.7059086127755,-9.7900005843855,12.7099994156145));
#2557=CARTESIAN_POINT('',(-10.5,-9.29289321881345,12.5));
#2558=CARTESIAN_POINT('Origin',(-10.75,-2.5,12.25));
#2559=CARTESIAN_POINT('',(-11.,-5.5,12.));
#2560=CARTESIAN_POINT('',(-10.5,-5.70710678118654,12.5));
#2561=CARTESIAN_POINT('',(-11.,-2.5,12.));
#2562=CARTESIAN_POINT('Origin',(-6.44822330470336,-1.30177669529664,12.25));
#2563=CARTESIAN_POINT('',(-10.,-4.5,12.));
#2564=CARTESIAN_POINT('',(-9.79289321881345,-5.,12.5));
#2565=CARTESIAN_POINT('',(-6.62499999999999,-1.125,12.));
#2566=CARTESIAN_POINT('Origin',(2.5,-4.75,12.25));
#2567=CARTESIAN_POINT('',(5.,-4.5,12.));
#2568=CARTESIAN_POINT('',(3.08333333333333,-2.58333333333333,10.0833333333333));
#2569=CARTESIAN_POINT('',(2.5,-4.5,12.));
#2570=CARTESIAN_POINT('Origin',(-10.5,-10.,7.5));
#2571=CARTESIAN_POINT('',(-11.,-9.5,7.5));
#2572=CARTESIAN_POINT('',(-11.,-9.5,7.5));
#2573=CARTESIAN_POINT('',(-10.,-10.5,7.5));
#2574=CARTESIAN_POINT('',(-10.375,-10.125,7.5));
#2575=CARTESIAN_POINT('',(-10.,-10.5,7.5));
#2576=CARTESIAN_POINT('Origin',(-11.,-5.,7.5));
#2577=CARTESIAN_POINT('',(-11.,-5.5,7.5));
#2578=CARTESIAN_POINT('',(-11.,-5.5,7.5));
#2579=CARTESIAN_POINT('',(-11.,8.,7.5));
#2580=CARTESIAN_POINT('Origin',(-10.5,-5.,7.5));
#2581=CARTESIAN_POINT('',(-10.,-4.5,7.5));
#2582=CARTESIAN_POINT('',(-10.,-4.5,7.5));
#2583=CARTESIAN_POINT('',(-6.62499999999999,-1.125,7.5));
#2584=CARTESIAN_POINT('Origin',(5.,-4.5,7.5));
#2585=CARTESIAN_POINT('',(5.,-4.5,7.5));
#2586=CARTESIAN_POINT('',(5.,-4.5,7.5));
#2587=CARTESIAN_POINT('',(2.5,-4.5,7.5));
#2588=CARTESIAN_POINT('Origin',(0.,0.,7.5));
#2589=CARTESIAN_POINT('',(5.,10.,7.5));
#2590=CARTESIAN_POINT('',(5.,11.,7.5));
#2591=CARTESIAN_POINT('',(6.,11.,7.5));
#2592=CARTESIAN_POINT('',(1.5,6.5,7.5));
#2593=CARTESIAN_POINT('',(10.,11.,7.5));
#2594=CARTESIAN_POINT('',(5.,11.,7.5));
#2595=CARTESIAN_POINT('',(11.,10.,7.5));
#2596=CARTESIAN_POINT('',(10.5,10.5,7.5));
#2597=CARTESIAN_POINT('',(11.,-9.5,7.5));
#2598=CARTESIAN_POINT('',(11.,-11.,7.5));
#2599=CARTESIAN_POINT('',(10.,-10.5,7.5));
#2600=CARTESIAN_POINT('',(10.375,-10.125,7.5));
#2601=CARTESIAN_POINT('',(-5.5,-10.5,7.5));
#2602=CARTESIAN_POINT('',(10.,7.5,7.5));
#2603=CARTESIAN_POINT('Origin',(8.,7.5,7.5));
#2604=CARTESIAN_POINT('Origin',(5.25,5.5,12.25));
#2605=CARTESIAN_POINT('',(5.,10.,12.));
#2606=CARTESIAN_POINT('',(5.,5.5,12.));
#2607=CARTESIAN_POINT('',(5.5,9.79289321881345,12.5));
#2608=CARTESIAN_POINT('Origin',(5.5,10.75,12.25));
#2609=CARTESIAN_POINT('',(10.,11.,12.));
#2610=CARTESIAN_POINT('',(9.79289321881345,10.5,12.5));
#2611=CARTESIAN_POINT('',(6.,11.,12.));
#2612=CARTESIAN_POINT('',(5.5,11.,12.));
#2613=CARTESIAN_POINT('',(6.,11.,12.));
#2614=CARTESIAN_POINT('Origin',(10.3232233047034,10.3232233047034,12.25));
#2615=CARTESIAN_POINT('',(11.,10.,12.));
#2616=CARTESIAN_POINT('',(10.5,9.79289321881345,12.5));
#2617=CARTESIAN_POINT('',(10.5,10.5,12.));
#2618=CARTESIAN_POINT('Origin',(10.75,-5.5,12.25));
#2619=CARTESIAN_POINT('',(11.,-9.5,12.));
#2620=CARTESIAN_POINT('',(10.5,-9.29289321881345,12.5));
#2621=CARTESIAN_POINT('',(11.,-5.5,12.));
#2622=CARTESIAN_POINT('Origin',(10.1982233047034,-9.94822330470337,12.25));
#2623=CARTESIAN_POINT('',(10.,-10.5,12.));
#2624=CARTESIAN_POINT('',(9.79289321881345,-10.,12.5));
#2625=CARTESIAN_POINT('',(10.375,-10.125,12.));
#2626=CARTESIAN_POINT('Origin',(-5.5,-10.25,12.25));
#2627=CARTESIAN_POINT('',(-5.5,-10.5,12.));
#2628=CARTESIAN_POINT('Origin',(1.67677669529664,6.32322330470336,12.25));
#2629=CARTESIAN_POINT('',(1.5,6.5,12.));
#2630=CARTESIAN_POINT('Origin',(5.,11.,7.5));
#2631=CARTESIAN_POINT('',(5.,10.,7.5));
#2632=CARTESIAN_POINT('Origin',(5.5,10.5,7.5));
#2633=CARTESIAN_POINT('',(6.,11.,7.5));
#2634=CARTESIAN_POINT('Origin',(11.,11.,7.5));
#2635=CARTESIAN_POINT('',(10.,11.,7.5));
#2636=CARTESIAN_POINT('Origin',(10.5,10.5,7.5));
#2637=CARTESIAN_POINT('',(11.,10.,7.5));
#2638=CARTESIAN_POINT('Origin',(11.,-11.,7.5));
#2639=CARTESIAN_POINT('',(11.,-9.5,7.5));
#2640=CARTESIAN_POINT('Origin',(10.5,-10.,7.5));
#2641=CARTESIAN_POINT('',(10.,-10.5,7.5));
#2642=CARTESIAN_POINT('Origin',(-11.,-10.5,7.5));
#2643=CARTESIAN_POINT('Origin',(8.,7.5,12.35));
#2644=CARTESIAN_POINT('',(10.,7.5,12.2));
#2645=CARTESIAN_POINT('Origin',(8.,7.5,12.2));
#2646=CARTESIAN_POINT('',(10.15,7.5,12.35));
#2647=CARTESIAN_POINT('Origin',(8.,7.5,12.5));
#2648=CARTESIAN_POINT('',(10.,7.5,12.5));
#2665=UNCERTAINTY_MEASURE_WITH_UNIT(LENGTH_MEASURE(0.01),#2677,
'DISTANCE_ACCURACY_VALUE',
'Maximum model space distance between geometric entities at asserted c
onnectivities');
#2666=UNCERTAINTY_MEASURE_WITH_UNIT(LENGTH_MEASURE(0.01),#2677,
'DISTANCE_ACCURACY_VALUE',
'Maximum model space distance between geometric entities at asserted c
onnectivities');
#2675=(
GEOMETRIC_REPRESENTATION_CONTEXT(3)
GLOBAL_UNCERTAINTY_ASSIGNED_CONTEXT((#2665))
GLOBAL_UNIT_ASSIGNED_CONTEXT((#2677,#2679,#2680))
REPRESENTATION_CONTEXT('','3D')
);
#2676=(
GEOMETRIC_REPRESENTATION_CONTEXT(3)
GLOBAL_UNCERTAINTY_ASSIGNED_CONTEXT((#2666))
GLOBAL_UNIT_ASSIGNED_CONTEXT((#2677,#2679,#2680))
REPRESENTATION_CONTEXT('','3D')
);
#2677=(
LENGTH_UNIT()
NAMED_UNIT(*)
SI_UNIT(.MILLI.,.METRE.)
);
#2679=(
NAMED_UNIT(*)
PLANE_ANGLE_UNIT()
SI_UNIT($,.RADIAN.)
);
#2680=(
NAMED_UNIT(*)
SI_UNIT($,.STERADIAN.)
SOLID_ANGLE_UNIT()
);
#2689=SHAPE_DEFINITION_REPRESENTATION(#2698,#2715);
#2698=PRODUCT_DEFINITION_SHAPE('',$,#2725);
#2715=SHAPE_REPRESENTATION('',(#1714),#2675);
#2716=PRODUCT_DEFINITION_CONTEXT('part definition',#2745,'design');
#2725=PRODUCT_DEFINITION('Top_Part','Top_part',#2734,#2716);
#2734=PRODUCT_DEFINITION_FORMATION('',$,#2755);
#2745=APPLICATION_CONTEXT(
'Core Data for Automotive Mechanical Design Process');
#2746=PRODUCT_CONTEXT('part definition',#2745,'mechanical');
#2755=PRODUCT('Top_Part','Top_part',$,(#2746));
#2757=PRESENTATION_STYLE_ASSIGNMENT((#2759));
#2759=SURFACE_STYLE_USAGE(.BOTH.,#2761);
#2761=SURFACE_SIDE_STYLE('',(#2763));
#2763=SURFACE_STYLE_FILL_AREA(#2765);
#2765=FILL_AREA_STYLE('Opaque(203,203,203)',(#2767));
#2767=FILL_AREA_STYLE_COLOUR('Opaque(203,203,203)',#2769);
#2769=COLOUR_RGB('Opaque(203,203,203)', 0.09019608, 0.27058824, 0.51372549);
ENDSEC;
END-ISO-10303-21;
